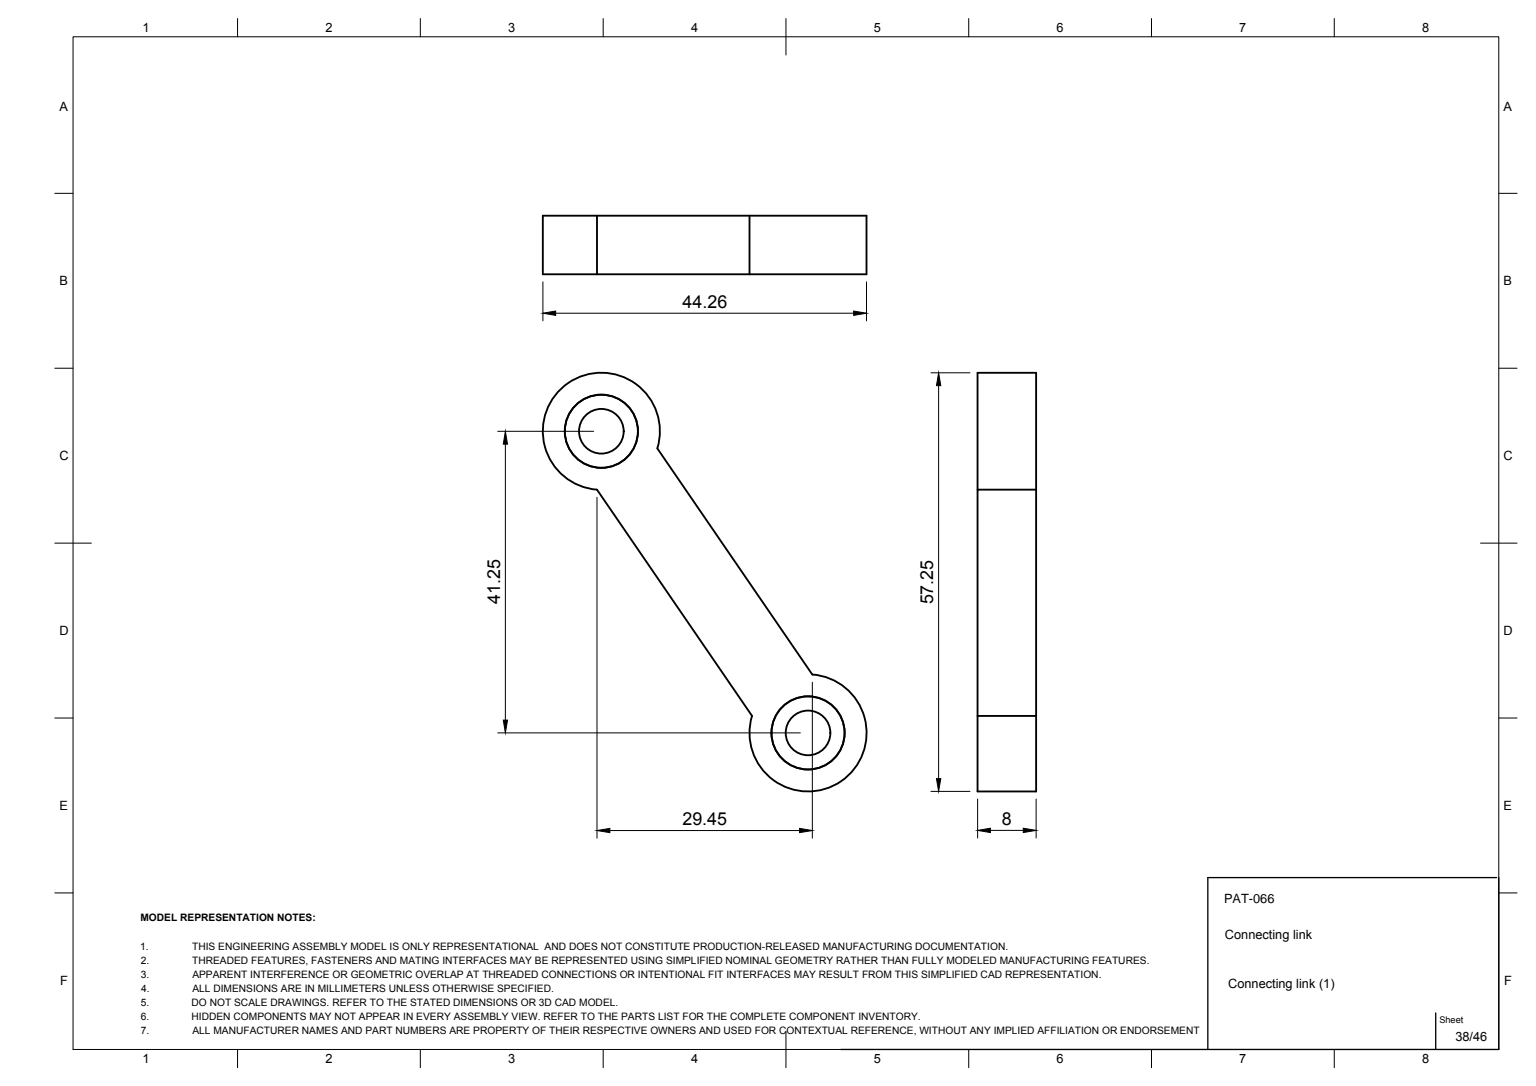
ISO-10303-21;
HEADER;
/* Generated by software containing ST-Developer
 * from STEP Tools, Inc. (www.steptools.com) 
 */

FILE_DESCRIPTION(
/* description */ ('Lever-operated bar clamp (toggle)'),
/* implementation_level */ '2;1');

FILE_NAME(
/* name */ 'Connecting link.step',
/* time_stamp */ '2026-10-28T03:25:02-07:00',
/* author */ (''),
/* organization */ (''),
/* preprocessor_version */ 'ST-DEVELOPER v20.2',
/* originating_system */ 'Autodesk Translation Framework v15.17.0.0',
/* authorisation */ '');

FILE_SCHEMA (('AUTOMOTIVE_DESIGN { 1 0 10303 214 3 1 1 }'));
ENDSEC;

DATA;
#10=MECHANICAL_DESIGN_GEOMETRIC_PRESENTATION_REPRESENTATION('',(#449),#12413);
#365=SHAPE_REPRESENTATION_RELATIONSHIP('SRR','None',#12608,#403);
#403=ADVANCED_BREP_SHAPE_REPRESENTATION('',(#492),#12405);
#449=STYLED_ITEM('',(#12862),#492);
#492=MANIFOLD_SOLID_BREP('Body1',#6612);
#636=FACE_BOUND('',#1781,.T.);
#637=FACE_BOUND('',#1782,.T.);
#638=FACE_BOUND('',#1786,.T.);
#639=FACE_BOUND('',#1787,.T.);
#847=PLANE('',#7784);
#848=PLANE('',#7785);
#849=PLANE('',#7787);
#850=PLANE('',#7790);
#1234=FACE_OUTER_BOUND('',#1776,.T.);
#1235=FACE_OUTER_BOUND('',#1777,.T.);
#1236=FACE_OUTER_BOUND('',#1778,.T.);
#1237=FACE_OUTER_BOUND('',#1779,.T.);
#1238=FACE_OUTER_BOUND('',#1780,.T.);
#1239=FACE_OUTER_BOUND('',#1783,.T.);
#1240=FACE_OUTER_BOUND('',#1784,.T.);
#1241=FACE_OUTER_BOUND('',#1785,.T.);
#1776=EDGE_LOOP('',(#5793,#5794,#5795,#5796));
#1777=EDGE_LOOP('',(#5797,#5798,#5799,#5800));
#1778=EDGE_LOOP('',(#5801,#5802,#5803,#5804));
#1779=EDGE_LOOP('',(#5805,#5806,#5807,#5808));
#1780=EDGE_LOOP('',(#5809,#5810,#5811,#5812));
#1781=EDGE_LOOP('',(#5813));
#1782=EDGE_LOOP('',(#5814));
#1783=EDGE_LOOP('',(#5815,#5816,#5817,#5818));
#1784=EDGE_LOOP('',(#5819,#5820,#5821,#5822));
#1785=EDGE_LOOP('',(#5823,#5824,#5825,#5826));
#1786=EDGE_LOOP('',(#5827));
#1787=EDGE_LOOP('',(#5828));
#2215=LINE('',#12031,#2656);
#2216=LINE('',#12037,#2657);
#2217=LINE('',#12042,#2658);
#2218=LINE('',#12046,#2659);
#2219=LINE('',#12050,#2660);
#2220=LINE('',#12052,#2661);
#2221=LINE('',#12053,#2662);
#2222=LINE('',#12056,#2663);
#2223=LINE('',#12060,#2664);
#2224=LINE('',#12061,#2665);
#2656=VECTOR('',#9734,0.5);
#2657=VECTOR('',#9741,0.5);
#2658=VECTOR('',#9746,1.);
#2659=VECTOR('',#9749,1.);
#2660=VECTOR('',#9754,1.);
#2661=VECTOR('',#9755,1.);
#2662=VECTOR('',#9756,1.);
#2663=VECTOR('',#9759,1.);
#2664=VECTOR('',#9764,1.);
#2665=VECTOR('',#9765,1.);
#3033=CIRCLE('',#7776,0.5);
#3034=CIRCLE('',#7777,0.5);
#3035=CIRCLE('',#7779,0.5);
#3036=CIRCLE('',#7780,0.5);
#3037=CIRCLE('',#7782,0.8);
#3038=CIRCLE('',#7783,0.8);
#3039=CIRCLE('',#7786,0.8);
#3040=CIRCLE('',#7789,0.8);
#3536=VERTEX_POINT('',#12028);
#3537=VERTEX_POINT('',#12030);
#3538=VERTEX_POINT('',#12034);
#3539=VERTEX_POINT('',#12036);
#3540=VERTEX_POINT('',#12040);
#3541=VERTEX_POINT('',#12041);
#3542=VERTEX_POINT('',#12043);
#3543=VERTEX_POINT('',#12045);
#3544=VERTEX_POINT('',#12049);
#3545=VERTEX_POINT('',#12051);
#3546=VERTEX_POINT('',#12055);
#3547=VERTEX_POINT('',#12059);
#4301=EDGE_CURVE('',#3536,#3536,#3033,.T.);
#4302=EDGE_CURVE('',#3536,#3537,#2215,.T.);
#4303=EDGE_CURVE('',#3537,#3537,#3034,.T.);
#4304=EDGE_CURVE('',#3538,#3538,#3035,.T.);
#4305=EDGE_CURVE('',#3538,#3539,#2216,.T.);
#4306=EDGE_CURVE('',#3539,#3539,#3036,.T.);
#4307=EDGE_CURVE('',#3540,#3541,#2217,.T.);
#4308=EDGE_CURVE('',#3542,#3540,#3037,.T.);
#4309=EDGE_CURVE('',#3543,#3542,#2218,.T.);
#4310=EDGE_CURVE('',#3543,#3541,#3038,.T.);
#4311=EDGE_CURVE('',#3541,#3544,#2219,.T.);
#4312=EDGE_CURVE('',#3545,#3544,#2220,.T.);
#4313=EDGE_CURVE('',#3540,#3545,#2221,.T.);
#4314=EDGE_CURVE('',#3546,#3543,#2222,.T.);
#4315=EDGE_CURVE('',#3544,#3546,#3039,.T.);
#4316=EDGE_CURVE('',#3547,#3542,#2223,.T.);
#4317=EDGE_CURVE('',#3546,#3547,#2224,.T.);
#4318=EDGE_CURVE('',#3545,#3547,#3040,.T.);
#5793=ORIENTED_EDGE('',*,*,#4301,.F.);
#5794=ORIENTED_EDGE('',*,*,#4302,.T.);
#5795=ORIENTED_EDGE('',*,*,#4303,.F.);
#5796=ORIENTED_EDGE('',*,*,#4302,.F.);
#5797=ORIENTED_EDGE('',*,*,#4304,.F.);
#5798=ORIENTED_EDGE('',*,*,#4305,.T.);
#5799=ORIENTED_EDGE('',*,*,#4306,.F.);
#5800=ORIENTED_EDGE('',*,*,#4305,.F.);
#5801=ORIENTED_EDGE('',*,*,#4307,.F.);
#5802=ORIENTED_EDGE('',*,*,#4308,.F.);
#5803=ORIENTED_EDGE('',*,*,#4309,.F.);
#5804=ORIENTED_EDGE('',*,*,#4310,.T.);
#5805=ORIENTED_EDGE('',*,*,#4307,.T.);
#5806=ORIENTED_EDGE('',*,*,#4311,.T.);
#5807=ORIENTED_EDGE('',*,*,#4312,.F.);
#5808=ORIENTED_EDGE('',*,*,#4313,.F.);
#5809=ORIENTED_EDGE('',*,*,#4310,.F.);
#5810=ORIENTED_EDGE('',*,*,#4314,.F.);
#5811=ORIENTED_EDGE('',*,*,#4315,.F.);
#5812=ORIENTED_EDGE('',*,*,#4311,.F.);
#5813=ORIENTED_EDGE('',*,*,#4301,.T.);
#5814=ORIENTED_EDGE('',*,*,#4304,.T.);
#5815=ORIENTED_EDGE('',*,*,#4309,.T.);
#5816=ORIENTED_EDGE('',*,*,#4316,.F.);
#5817=ORIENTED_EDGE('',*,*,#4317,.F.);
#5818=ORIENTED_EDGE('',*,*,#4314,.T.);
#5819=ORIENTED_EDGE('',*,*,#4312,.T.);
#5820=ORIENTED_EDGE('',*,*,#4315,.T.);
#5821=ORIENTED_EDGE('',*,*,#4317,.T.);
#5822=ORIENTED_EDGE('',*,*,#4318,.F.);
#5823=ORIENTED_EDGE('',*,*,#4313,.T.);
#5824=ORIENTED_EDGE('',*,*,#4318,.T.);
#5825=ORIENTED_EDGE('',*,*,#4316,.T.);
#5826=ORIENTED_EDGE('',*,*,#4308,.T.);
#5827=ORIENTED_EDGE('',*,*,#4303,.T.);
#5828=ORIENTED_EDGE('',*,*,#4306,.T.);
#6146=CYLINDRICAL_SURFACE('',#7775,0.5);
#6147=CYLINDRICAL_SURFACE('',#7778,0.5);
#6148=CYLINDRICAL_SURFACE('',#7781,0.8);
#6149=CYLINDRICAL_SURFACE('',#7788,0.8);
#6509=ADVANCED_FACE('',(#1234),#6146,.F.);
#6510=ADVANCED_FACE('',(#1235),#6147,.F.);
#6511=ADVANCED_FACE('',(#1236),#6148,.T.);
#6512=ADVANCED_FACE('',(#1237),#847,.T.);
#6513=ADVANCED_FACE('',(#1238,#636,#637),#848,.F.);
#6514=ADVANCED_FACE('',(#1239),#849,.T.);
#6515=ADVANCED_FACE('',(#1240),#6149,.T.);
#6516=ADVANCED_FACE('',(#1241,#638,#639),#850,.T.);
#6612=CLOSED_SHELL('',(#6509,#6510,#6511,#6512,#6513,#6514,#6515,#6516));
#7774=AXIS2_PLACEMENT_3D('',#12026,#9728,#9729);
#7775=AXIS2_PLACEMENT_3D('',#12027,#9730,#9731);
#7776=AXIS2_PLACEMENT_3D('',#12029,#9732,#9733);
#7777=AXIS2_PLACEMENT_3D('',#12032,#9735,#9736);
#7778=AXIS2_PLACEMENT_3D('',#12033,#9737,#9738);
#7779=AXIS2_PLACEMENT_3D('',#12035,#9739,#9740);
#7780=AXIS2_PLACEMENT_3D('',#12038,#9742,#9743);
#7781=AXIS2_PLACEMENT_3D('',#12039,#9744,#9745);
#7782=AXIS2_PLACEMENT_3D('',#12044,#9747,#9748);
#7783=AXIS2_PLACEMENT_3D('',#12047,#9750,#9751);
#7784=AXIS2_PLACEMENT_3D('',#12048,#9752,#9753);
#7785=AXIS2_PLACEMENT_3D('',#12054,#9757,#9758);
#7786=AXIS2_PLACEMENT_3D('',#12057,#9760,#9761);
#7787=AXIS2_PLACEMENT_3D('',#12058,#9762,#9763);
#7788=AXIS2_PLACEMENT_3D('',#12062,#9766,#9767);
#7789=AXIS2_PLACEMENT_3D('',#12063,#9768,#9769);
#7790=AXIS2_PLACEMENT_3D('',#12064,#9770,#9771);
#9728=DIRECTION('axis',(0.,0.,1.));
#9729=DIRECTION('refdir',(1.,0.,0.));
#9730=DIRECTION('center_axis',(0.,1.,0.));
#9731=DIRECTION('ref_axis',(1.,0.,0.));
#9732=DIRECTION('center_axis',(0.,1.,0.));
#9733=DIRECTION('ref_axis',(1.,0.,0.));
#9734=DIRECTION('',(0.,1.,0.));
#9735=DIRECTION('center_axis',(0.,-1.,0.));
#9736=DIRECTION('ref_axis',(1.,0.,0.));
#9737=DIRECTION('center_axis',(0.,1.,0.));
#9738=DIRECTION('ref_axis',(1.,0.,0.));
#9739=DIRECTION('center_axis',(0.,1.,0.));
#9740=DIRECTION('ref_axis',(1.,0.,0.));
#9741=DIRECTION('',(0.,1.,0.));
#9742=DIRECTION('center_axis',(0.,-1.,0.));
#9743=DIRECTION('ref_axis',(1.,0.,0.));
#9744=DIRECTION('center_axis',(0.,1.,0.));
#9745=DIRECTION('ref_axis',(0.565264218607056,0.,-0.824909912149536));
#9746=DIRECTION('',(0.,-1.,0.));
#9747=DIRECTION('center_axis',(0.,1.,0.));
#9748=DIRECTION('ref_axis',(1.,0.,0.));
#9749=DIRECTION('',(0.,1.,0.));
#9750=DIRECTION('center_axis',(0.,1.,0.));
#9751=DIRECTION('ref_axis',(1.,0.,0.));
#9752=DIRECTION('center_axis',(-0.824909912149536,0.,-0.565264218607055));
#9753=DIRECTION('ref_axis',(-0.565264218607055,0.,0.824909912149537));
#9754=DIRECTION('',(-0.565264218607055,0.,0.824909912149537));
#9755=DIRECTION('',(0.,-1.,0.));
#9756=DIRECTION('',(-0.565264218607055,0.,0.824909912149537));
#9757=DIRECTION('center_axis',(0.,1.,0.));
#9758=DIRECTION('ref_axis',(1.,0.,0.));
#9759=DIRECTION('',(0.565264218607055,0.,-0.824909912149537));
#9760=DIRECTION('center_axis',(0.,1.,0.));
#9761=DIRECTION('ref_axis',(1.,0.,0.));
#9762=DIRECTION('center_axis',(0.824909912149536,0.,0.565264218607055));
#9763=DIRECTION('ref_axis',(0.565264218607055,0.,-0.824909912149537));
#9764=DIRECTION('',(0.565264218607055,0.,-0.824909912149537));
#9765=DIRECTION('',(0.,1.,0.));
#9766=DIRECTION('center_axis',(0.,1.,0.));
#9767=DIRECTION('ref_axis',(-0.565264218607055,0.,0.824909912149536));
#9768=DIRECTION('center_axis',(0.,1.,0.));
#9769=DIRECTION('ref_axis',(1.,0.,0.));
#9770=DIRECTION('center_axis',(0.,1.,0.));
#9771=DIRECTION('ref_axis',(1.,0.,0.));
#12026=CARTESIAN_POINT('',(0.,0.,0.));
#12027=CARTESIAN_POINT('Origin',(-2.82632109303527,-5.6,8.79263101785268));
#12028=CARTESIAN_POINT('',(-3.32632109303527,-5.5,8.79263101785268));
#12029=CARTESIAN_POINT('Origin',(-2.82632109303527,-5.5,8.79263101785268));
#12030=CARTESIAN_POINT('',(-3.32632109303527,-4.7,8.79263101785268));
#12031=CARTESIAN_POINT('',(-3.32632109303527,-5.6,8.79263101785268));
#12032=CARTESIAN_POINT('Origin',(-2.82632109303527,-4.7,8.79263101785268));
#12033=CARTESIAN_POINT('Origin',(0.,-5.6,4.668081457105));
#12034=CARTESIAN_POINT('',(-0.5,-5.5,4.668081457105));
#12035=CARTESIAN_POINT('Origin',(0.,-5.5,4.668081457105));
#12036=CARTESIAN_POINT('',(-0.5,-4.7,4.668081457105));
#12037=CARTESIAN_POINT('',(-0.5,-5.6,4.668081457105));
#12038=CARTESIAN_POINT('Origin',(0.,-4.7,4.668081457105));
#12039=CARTESIAN_POINT('Origin',(0.,-5.5,4.668081457105));
#12040=CARTESIAN_POINT('',(-0.765462347451497,-4.7,4.90060542282476));
#12041=CARTESIAN_POINT('',(-0.765462347451497,-5.5,4.90060542282476));
#12042=CARTESIAN_POINT('',(-0.765462347451497,-5.5,4.90060542282476));
#12043=CARTESIAN_POINT('',(0.059447564698039,-4.7,5.46586964143181));
#12044=CARTESIAN_POINT('Origin',(0.,-4.7,4.668081457105));
#12045=CARTESIAN_POINT('',(0.059447564698039,-5.5,5.46586964143181));
#12046=CARTESIAN_POINT('',(0.059447564698039,-5.5,5.46586964143181));
#12047=CARTESIAN_POINT('Origin',(0.,-5.5,4.668081457105));
#12048=CARTESIAN_POINT('Origin',(-0.412454956074768,-5.5,4.38544934780147));
#12049=CARTESIAN_POINT('',(-2.88576865773331,-5.5,7.99484283352587));
#12050=CARTESIAN_POINT('',(-0.412454956074768,-5.5,4.38544934780147));
#12051=CARTESIAN_POINT('',(-2.88576865773331,-4.7,7.99484283352587));
#12052=CARTESIAN_POINT('',(-2.88576865773331,-5.5,7.99484283352587));
#12053=CARTESIAN_POINT('',(-0.412454956074768,-4.7,4.38544934780147));
#12054=CARTESIAN_POINT('Origin',(-2.82632109303527,-5.5,8.79263101785268));
#12055=CARTESIAN_POINT('',(-2.06085874558378,-5.5,8.56010705213293));
#12056=CARTESIAN_POINT('',(-2.4138661369605,-5.5,9.07526312715621));
#12057=CARTESIAN_POINT('Origin',(-2.82632109303527,-5.5,8.79263101785268));
#12058=CARTESIAN_POINT('Origin',(-2.4138661369605,-5.5,9.07526312715621));
#12059=CARTESIAN_POINT('',(-2.06085874558378,-4.7,8.56010705213293));
#12060=CARTESIAN_POINT('',(-2.4138661369605,-4.7,9.07526312715621));
#12061=CARTESIAN_POINT('',(-2.06085874558378,-5.5,8.56010705213293));
#12062=CARTESIAN_POINT('Origin',(-2.82632109303527,-5.5,8.79263101785268));
#12063=CARTESIAN_POINT('Origin',(-2.82632109303527,-4.7,8.79263101785268));
#12064=CARTESIAN_POINT('Origin',(-2.82632109303527,-4.7,8.79263101785268));
#12359=UNCERTAINTY_MEASURE_WITH_UNIT(LENGTH_MEASURE(0.001),#12414,
'DISTANCE_ACCURACY_VALUE',
'Maximum model space distance between geometric entities at asserted c
onnectivities');
#12367=UNCERTAINTY_MEASURE_WITH_UNIT(LENGTH_MEASURE(0.001),#12414,
'DISTANCE_ACCURACY_VALUE',
'Maximum model space distance between geometric entities at asserted c
onnectivities');
#12405=(
GEOMETRIC_REPRESENTATION_CONTEXT(3)
GLOBAL_UNCERTAINTY_ASSIGNED_CONTEXT((#12359))
GLOBAL_UNIT_ASSIGNED_CONTEXT((#12414,#12416,#12417))
REPRESENTATION_CONTEXT('','3D')
);
#12413=(
GEOMETRIC_REPRESENTATION_CONTEXT(3)
GLOBAL_UNCERTAINTY_ASSIGNED_CONTEXT((#12367))
GLOBAL_UNIT_ASSIGNED_CONTEXT((#12414,#12416,#12417))
REPRESENTATION_CONTEXT('','3D')
);
#12414=(
LENGTH_UNIT()
NAMED_UNIT(*)
SI_UNIT(.CENTI.,.METRE.)
);
#12416=(
NAMED_UNIT(*)
PLANE_ANGLE_UNIT()
SI_UNIT($,.RADIAN.)
);
#12417=(
NAMED_UNIT(*)
SI_UNIT($,.STERADIAN.)
SOLID_ANGLE_UNIT()
);
#12455=SHAPE_DEFINITION_REPRESENTATION(#12552,#12608);
#12552=PRODUCT_DEFINITION_SHAPE('',$,#12654);
#12608=SHAPE_REPRESENTATION('',(#7774),#12405);
#12616=PRODUCT_DEFINITION_CONTEXT('part definition',#12753,'design');
#12654=PRODUCT_DEFINITION('Connecting link','Connecting link',#12699,
#12616);
#12699=PRODUCT_DEFINITION_FORMATION('',$,#12792);
#12753=APPLICATION_CONTEXT(
'Core Data for Automotive Mechanical Design Process');
#12754=PRODUCT_CONTEXT('part definition',#12753,'mechanical');
#12792=PRODUCT('Connecting link','Connecting link','Connecting link',
(#12754));
#12856=COLOUR_RGB('Sky Blue',0.24,0.69,0.87);
#12857=FILL_AREA_STYLE_COLOUR('',#12856);
#12858=FILL_AREA_STYLE('',(#12857));
#12859=SURFACE_STYLE_FILL_AREA(#12858);
#12860=SURFACE_SIDE_STYLE('',(#12859));
#12861=SURFACE_STYLE_USAGE(.BOTH.,#12860);
#12862=PRESENTATION_STYLE_ASSIGNMENT((#12861));
ENDSEC;
END-ISO-10303-21;
